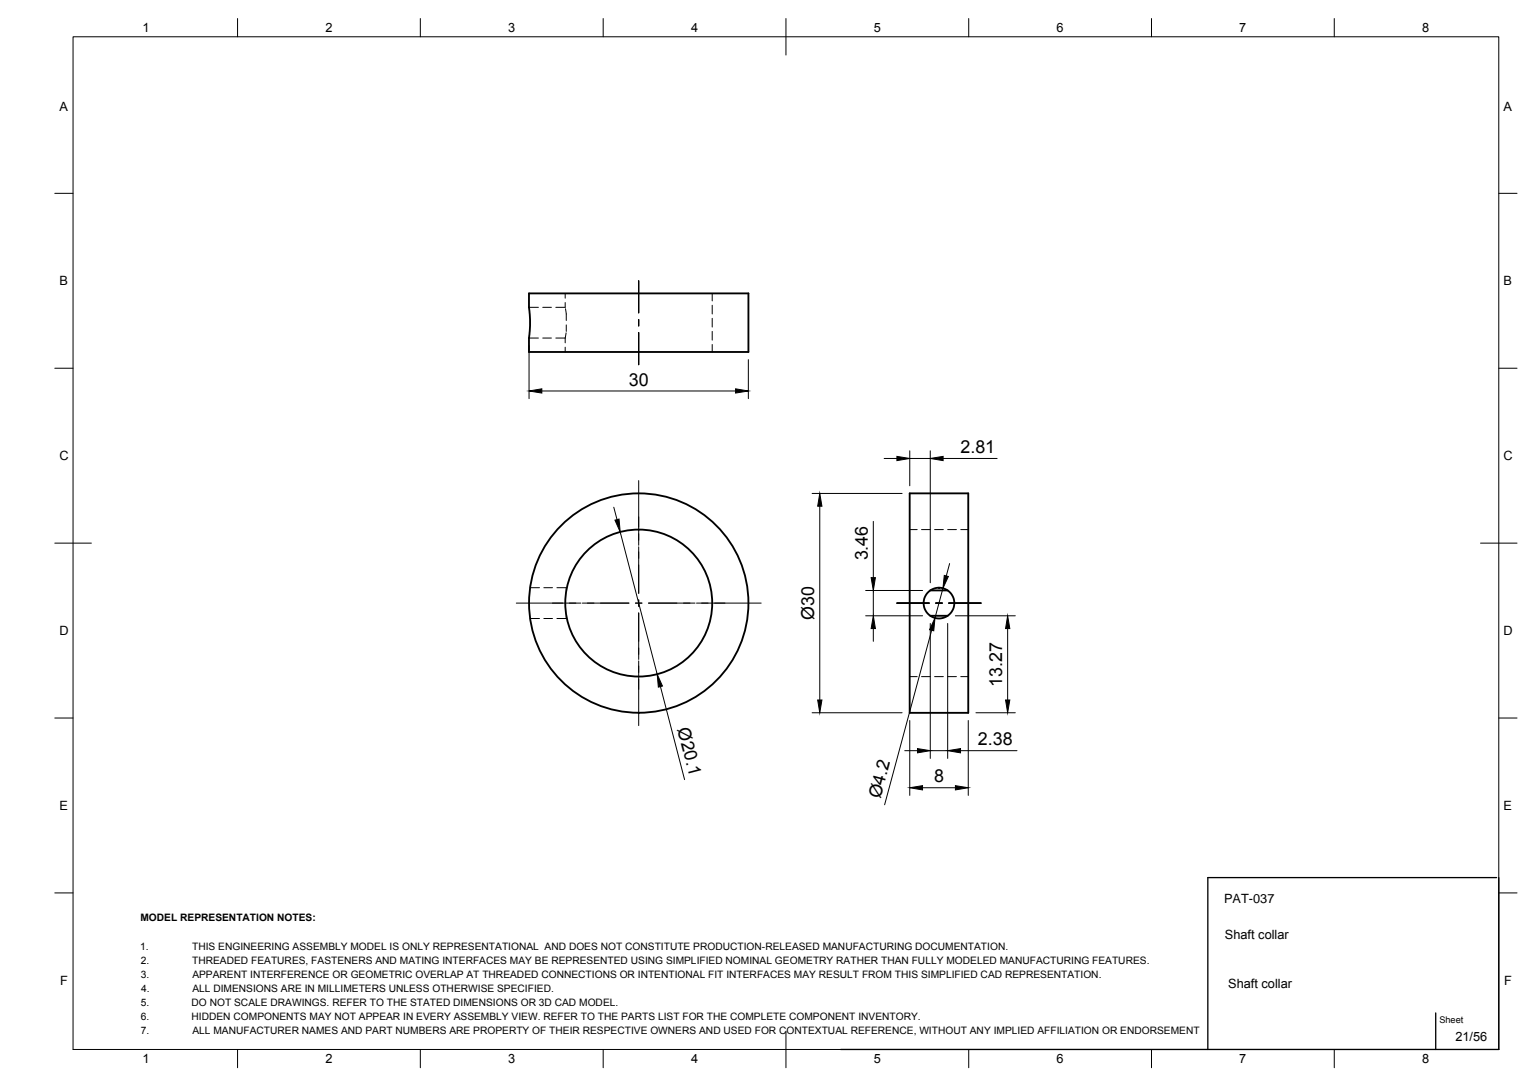
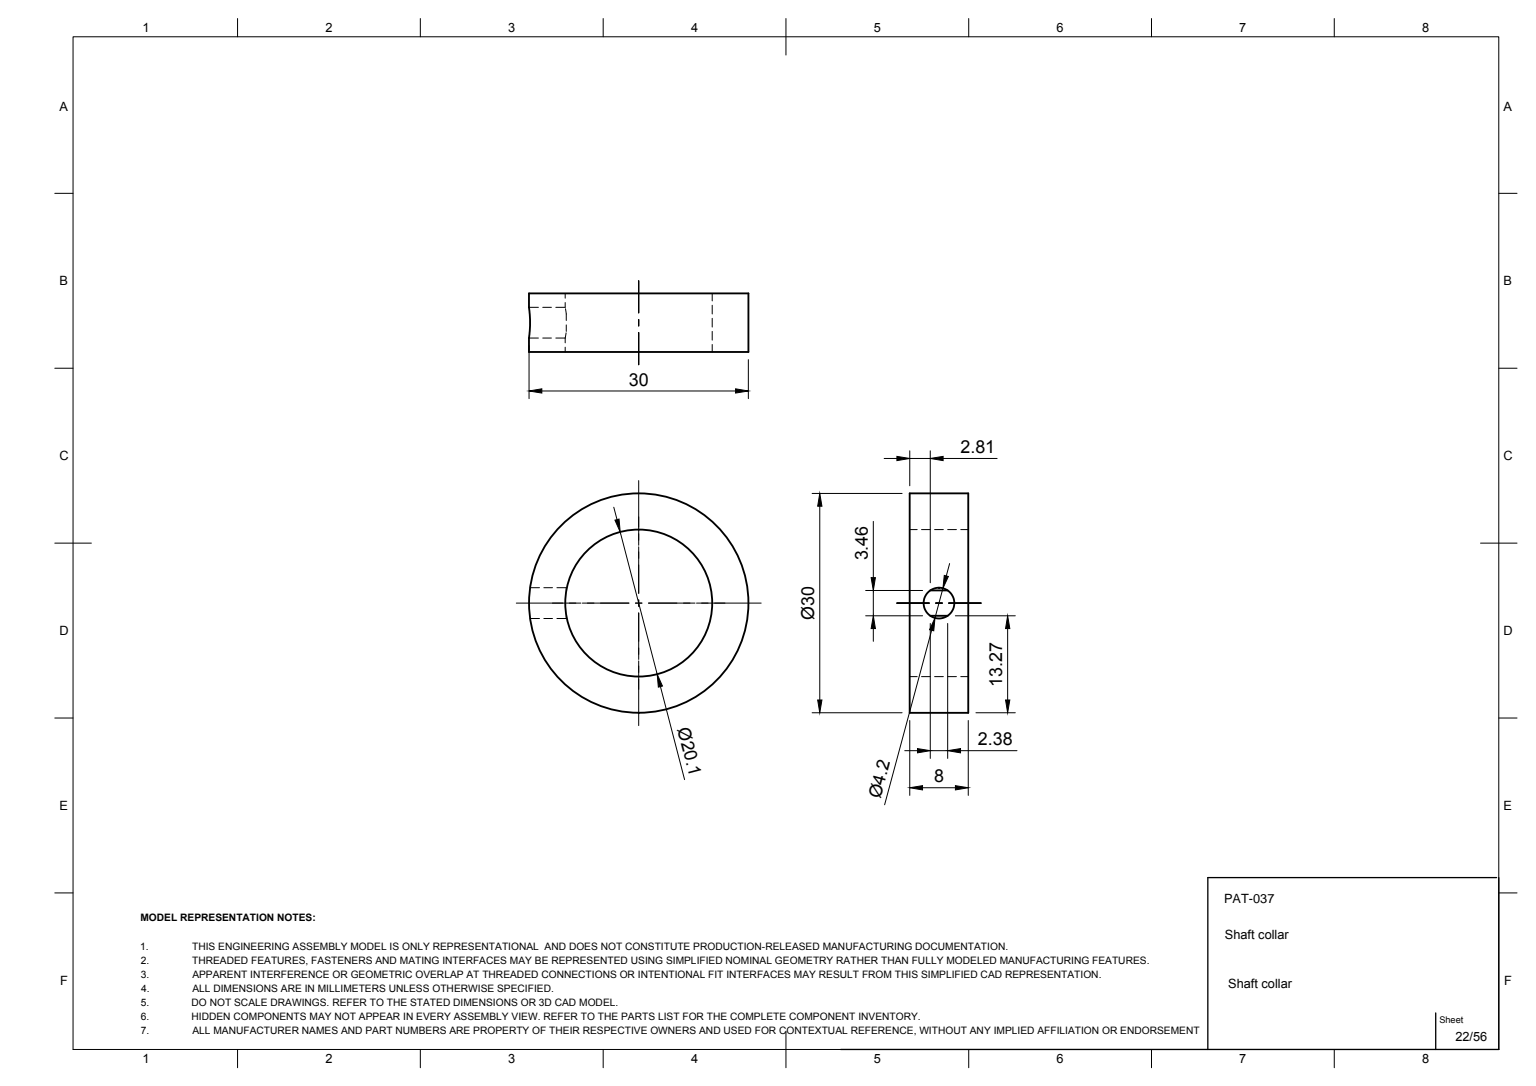
ISO-10303-21;
HEADER;
/* Generated by software containing ST-Developer
 * from STEP Tools, Inc. (www.steptools.com) 
 */

FILE_DESCRIPTION(
/* description */ ('Flywheel Crank-Slider'),
/* implementation_level */ '2;1');

FILE_NAME(
/* name */ 'Shaft collar.step',
/* time_stamp */ '2026-10-28T03:23:13-07:00',
/* author */ (''),
/* organization */ (''),
/* preprocessor_version */ 'ST-DEVELOPER v20.2',
/* originating_system */ 'Autodesk Translation Framework v15.17.0.0',
/* authorisation */ '');

FILE_SCHEMA (('AUTOMOTIVE_DESIGN { 1 0 10303 214 3 1 1 }'));
ENDSEC;

DATA;
#10=MECHANICAL_DESIGN_GEOMETRIC_PRESENTATION_REPRESENTATION('',(#691),#17322);
#481=B_SPLINE_CURVE_WITH_KNOTS('',3,(#15442,#15443,#15444,#15445,#15446,
#15447,#15448,#15449,#15450,#15451,#15452,#15453,#15454,#15455),
 .UNSPECIFIED.,.F.,.F.,(4,2,2,2,2,2,4),(0.756005737987026,0.793568827564645,
0.8729225200542,0.952276212543755,1.03162990503331,1.11098359752287,1.14854668710048),
 .UNSPECIFIED.);
#482=B_SPLINE_CURVE_WITH_KNOTS('',3,(#15461,#15462,#15463,#15464,#15465,
#15466,#15467,#15468,#15469,#15470,#15471,#15472,#15473,#15474,#15475,#15476,
#15477,#15478),.UNSPECIFIED.,.F.,.F.,(4,2,2,2,2,2,2,2,4),(0.,0.0792165807733624,
0.158433161546725,0.23764869707457,0.316864232602414,0.396079768130259,
0.475295303658103,0.554511884431466,0.633728465204828),.UNSPECIFIED.);
#483=B_SPLINE_CURVE_WITH_KNOTS('',3,(#15479,#15480,#15481,#15482,#15483,
#15484,#15485,#15486,#15487,#15488,#15489,#15490,#15491,#15492,#15493,#15494,
#15495,#15496),.UNSPECIFIED.,.F.,.F.,(4,2,2,2,2,2,2,2,4),(0.633728465204828,
0.712945045978191,0.792161626751553,0.871377162279398,0.950592697807242,
1.02980823333509,1.10902376886293,1.18824034963629,1.26745693040966),
 .UNSPECIFIED.);
#484=B_SPLINE_CURVE_WITH_KNOTS('',3,(#15499,#15500,#15501,#15502,#15503,
#15504,#15505,#15506,#15507,#15508,#15509,#15510,#15511,#15512),
 .UNSPECIFIED.,.F.,.F.,(4,2,2,2,2,2,4),(0.121154929624522,0.158718019202141,
0.238071711691697,0.317425404181252,0.396779096670807,0.476132789160362,
0.513695878737981),.UNSPECIFIED.);
#586=SHAPE_REPRESENTATION_RELATIONSHIP('SRR','None',#17584,#638);
#638=ADVANCED_BREP_SHAPE_REPRESENTATION('',(#748),#17288);
#691=STYLED_ITEM('',(#17931),#748);
#748=MANIFOLD_SOLID_BREP('Body1',#9073);
#908=FACE_BOUND('',#2264,.T.);
#909=FACE_BOUND('',#2266,.T.);
#910=FACE_BOUND('',#2268,.T.);
#911=FACE_BOUND('',#2270,.T.);
#1181=PLANE('',#10198);
#1182=PLANE('',#10203);
#1183=PLANE('',#10210);
#1184=PLANE('',#10211);
#1602=FACE_OUTER_BOUND('',#2260,.T.);
#1603=FACE_OUTER_BOUND('',#2261,.T.);
#1604=FACE_OUTER_BOUND('',#2262,.T.);
#1605=FACE_OUTER_BOUND('',#2263,.T.);
#1606=FACE_OUTER_BOUND('',#2265,.T.);
#1607=FACE_OUTER_BOUND('',#2267,.T.);
#1608=FACE_OUTER_BOUND('',#2269,.T.);
#2260=EDGE_LOOP('',(#7308,#7309));
#2261=EDGE_LOOP('',(#7310,#7311,#7312,#7313,#7314,#7315,#7316,#7317,#7318));
#2262=EDGE_LOOP('',(#7319,#7320,#7321));
#2263=EDGE_LOOP('',(#7322,#7323,#7324,#7325));
#2264=EDGE_LOOP('',(#7326,#7327,#7328,#7329));
#2265=EDGE_LOOP('',(#7330,#7331,#7332,#7333));
#2266=EDGE_LOOP('',(#7334,#7335));
#2267=EDGE_LOOP('',(#7336));
#2268=EDGE_LOOP('',(#7337));
#2269=EDGE_LOOP('',(#7338));
#2270=EDGE_LOOP('',(#7339));
#2983=LINE('',#15438,#3594);
#2984=LINE('',#15459,#3595);
#2985=LINE('',#15514,#3596);
#2986=LINE('',#15519,#3597);
#2987=LINE('',#15525,#3598);
#3594=VECTOR('',#12225,1.);
#3595=VECTOR('',#12232,0.21);
#3596=VECTOR('',#12237,1.);
#3597=VECTOR('',#12242,1.005);
#3598=VECTOR('',#12249,1.5);
#4040=CIRCLE('',#10199,0.21);
#4041=CIRCLE('',#10201,0.21);
#4042=CIRCLE('',#10202,0.21);
#4043=CIRCLE('',#10205,1.005);
#4044=CIRCLE('',#10206,1.005);
#4045=CIRCLE('',#10208,1.5);
#4046=CIRCLE('',#10209,1.5);
#4669=VERTEX_POINT('',#15436);
#4670=VERTEX_POINT('',#15437);
#4671=VERTEX_POINT('',#15441);
#4672=VERTEX_POINT('',#15456);
#4673=VERTEX_POINT('',#15458);
#4674=VERTEX_POINT('',#15460);
#4675=VERTEX_POINT('',#15497);
#4676=VERTEX_POINT('',#15516);
#4677=VERTEX_POINT('',#15518);
#4678=VERTEX_POINT('',#15522);
#4679=VERTEX_POINT('',#15524);
#5611=EDGE_CURVE('',#4669,#4670,#2983,.T.);
#5612=EDGE_CURVE('',#4669,#4670,#4040,.T.);
#5613=EDGE_CURVE('',#4671,#4669,#481,.T.);
#5614=EDGE_CURVE('',#4672,#4671,#4041,.T.);
#5615=EDGE_CURVE('',#4672,#4673,#2984,.T.);
#5616=EDGE_CURVE('',#4674,#4673,#482,.T.);
#5617=EDGE_CURVE('',#4673,#4674,#483,.T.);
#5618=EDGE_CURVE('',#4675,#4672,#4042,.T.);
#5619=EDGE_CURVE('',#4670,#4675,#484,.T.);
#5620=EDGE_CURVE('',#4675,#4671,#2985,.T.);
#5621=EDGE_CURVE('',#4676,#4676,#4043,.T.);
#5622=EDGE_CURVE('',#4676,#4677,#2986,.T.);
#5623=EDGE_CURVE('',#4677,#4677,#4044,.T.);
#5624=EDGE_CURVE('',#4678,#4678,#4045,.T.);
#5625=EDGE_CURVE('',#4678,#4679,#2987,.T.);
#5626=EDGE_CURVE('',#4679,#4679,#4046,.T.);
#7308=ORIENTED_EDGE('',*,*,#5611,.F.);
#7309=ORIENTED_EDGE('',*,*,#5612,.T.);
#7310=ORIENTED_EDGE('',*,*,#5613,.F.);
#7311=ORIENTED_EDGE('',*,*,#5614,.F.);
#7312=ORIENTED_EDGE('',*,*,#5615,.T.);
#7313=ORIENTED_EDGE('',*,*,#5616,.F.);
#7314=ORIENTED_EDGE('',*,*,#5617,.F.);
#7315=ORIENTED_EDGE('',*,*,#5615,.F.);
#7316=ORIENTED_EDGE('',*,*,#5618,.F.);
#7317=ORIENTED_EDGE('',*,*,#5619,.F.);
#7318=ORIENTED_EDGE('',*,*,#5612,.F.);
#7319=ORIENTED_EDGE('',*,*,#5620,.F.);
#7320=ORIENTED_EDGE('',*,*,#5618,.T.);
#7321=ORIENTED_EDGE('',*,*,#5614,.T.);
#7322=ORIENTED_EDGE('',*,*,#5621,.F.);
#7323=ORIENTED_EDGE('',*,*,#5622,.T.);
#7324=ORIENTED_EDGE('',*,*,#5623,.T.);
#7325=ORIENTED_EDGE('',*,*,#5622,.F.);
#7326=ORIENTED_EDGE('',*,*,#5619,.T.);
#7327=ORIENTED_EDGE('',*,*,#5620,.T.);
#7328=ORIENTED_EDGE('',*,*,#5613,.T.);
#7329=ORIENTED_EDGE('',*,*,#5611,.T.);
#7330=ORIENTED_EDGE('',*,*,#5624,.F.);
#7331=ORIENTED_EDGE('',*,*,#5625,.T.);
#7332=ORIENTED_EDGE('',*,*,#5626,.T.);
#7333=ORIENTED_EDGE('',*,*,#5625,.F.);
#7334=ORIENTED_EDGE('',*,*,#5616,.T.);
#7335=ORIENTED_EDGE('',*,*,#5617,.T.);
#7336=ORIENTED_EDGE('',*,*,#5624,.T.);
#7337=ORIENTED_EDGE('',*,*,#5621,.T.);
#7338=ORIENTED_EDGE('',*,*,#5626,.F.);
#7339=ORIENTED_EDGE('',*,*,#5623,.F.);
#8424=CYLINDRICAL_SURFACE('',#10200,0.21);
#8425=CYLINDRICAL_SURFACE('',#10204,1.005);
#8426=CYLINDRICAL_SURFACE('',#10207,1.5);
#8793=ADVANCED_FACE('',(#1602),#1181,.T.);
#8794=ADVANCED_FACE('',(#1603),#8424,.F.);
#8795=ADVANCED_FACE('',(#1604),#1182,.T.);
#8796=ADVANCED_FACE('',(#1605,#908),#8425,.F.);
#8797=ADVANCED_FACE('',(#1606,#909),#8426,.T.);
#8798=ADVANCED_FACE('',(#1607,#910),#1183,.T.);
#8799=ADVANCED_FACE('',(#1608,#911),#1184,.F.);
#9073=CLOSED_SHELL('',(#8793,#8794,#8795,#8796,#8797,#8798,#8799));
#10197=AXIS2_PLACEMENT_3D('',#15434,#12221,#12222);
#10198=AXIS2_PLACEMENT_3D('',#15435,#12223,#12224);
#10199=AXIS2_PLACEMENT_3D('',#15439,#12226,#12227);
#10200=AXIS2_PLACEMENT_3D('',#15440,#12228,#12229);
#10201=AXIS2_PLACEMENT_3D('',#15457,#12230,#12231);
#10202=AXIS2_PLACEMENT_3D('',#15498,#12233,#12234);
#10203=AXIS2_PLACEMENT_3D('',#15513,#12235,#12236);
#10204=AXIS2_PLACEMENT_3D('',#15515,#12238,#12239);
#10205=AXIS2_PLACEMENT_3D('',#15517,#12240,#12241);
#10206=AXIS2_PLACEMENT_3D('',#15520,#12243,#12244);
#10207=AXIS2_PLACEMENT_3D('',#15521,#12245,#12246);
#10208=AXIS2_PLACEMENT_3D('',#15523,#12247,#12248);
#10209=AXIS2_PLACEMENT_3D('',#15526,#12250,#12251);
#10210=AXIS2_PLACEMENT_3D('',#15527,#12252,#12253);
#10211=AXIS2_PLACEMENT_3D('',#15528,#12254,#12255);
#12221=DIRECTION('axis',(0.,0.,1.));
#12222=DIRECTION('refdir',(1.,0.,0.));
#12223=DIRECTION('center_axis',(0.,0.,1.));
#12224=DIRECTION('ref_axis',(1.,0.,0.));
#12225=DIRECTION('',(0.,1.,0.));
#12226=DIRECTION('center_axis',(0.,0.,1.));
#12227=DIRECTION('ref_axis',(1.,0.,0.));
#12228=DIRECTION('center_axis',(0.,0.,1.));
#12229=DIRECTION('ref_axis',(1.,0.,0.));
#12230=DIRECTION('center_axis',(0.,0.,1.));
#12231=DIRECTION('ref_axis',(1.,0.,0.));
#12232=DIRECTION('',(0.,0.,1.));
#12233=DIRECTION('center_axis',(0.,0.,1.));
#12234=DIRECTION('ref_axis',(1.,0.,0.));
#12235=DIRECTION('center_axis',(0.,0.,1.));
#12236=DIRECTION('ref_axis',(1.,0.,0.));
#12237=DIRECTION('',(0.,-1.,0.));
#12238=DIRECTION('center_axis',(0.,1.,0.));
#12239=DIRECTION('ref_axis',(1.,0.,0.));
#12240=DIRECTION('center_axis',(0.,-1.,0.));
#12241=DIRECTION('ref_axis',(1.,0.,0.));
#12242=DIRECTION('',(0.,-1.,0.));
#12243=DIRECTION('center_axis',(0.,-1.,0.));
#12244=DIRECTION('ref_axis',(1.,0.,0.));
#12245=DIRECTION('center_axis',(0.,1.,0.));
#12246=DIRECTION('ref_axis',(1.,0.,0.));
#12247=DIRECTION('center_axis',(0.,1.,0.));
#12248=DIRECTION('ref_axis',(1.,0.,0.));
#12249=DIRECTION('',(0.,-1.,0.));
#12250=DIRECTION('center_axis',(0.,1.,0.));
#12251=DIRECTION('ref_axis',(1.,0.,0.));
#12252=DIRECTION('center_axis',(0.,1.,0.));
#12253=DIRECTION('ref_axis',(1.,0.,0.));
#12254=DIRECTION('center_axis',(0.,1.,0.));
#12255=DIRECTION('ref_axis',(1.,0.,0.));
#15434=CARTESIAN_POINT('',(0.,0.,0.));
#15435=CARTESIAN_POINT('Origin',(0.,-17.05,10.99));
#15436=CARTESIAN_POINT('',(0.172988438920051,-17.1690588089979,10.99));
#15437=CARTESIAN_POINT('',(0.172988438920051,-16.9309411910021,10.99));
#15438=CARTESIAN_POINT('',(0.172988438920051,-17.45,10.99));
#15439=CARTESIAN_POINT('Origin',(0.,-17.05,10.99));
#15440=CARTESIAN_POINT('Origin',(0.,-17.05,10.99));
#15441=CARTESIAN_POINT('',(-0.172988438920051,-17.1690588089979,10.99));
#15442=CARTESIAN_POINT('Ctrl Pts',(-0.172988438920051,-17.1690588089979,
10.99));
#15443=CARTESIAN_POINT('Ctrl Pts',(-0.165594865311311,-17.1798014223953,
10.9912919219764));
#15444=CARTESIAN_POINT('Ctrl Pts',(-0.157297138725604,-17.1896877093727,
10.992653949439));
#15445=CARTESIAN_POINT('Ctrl Pts',(-0.129892073845076,-17.2170927742533,
10.9967480843909));
#15446=CARTESIAN_POINT('Ctrl Pts',(-0.106330167759284,-17.233242056333,
10.9996958932764));
#15447=CARTESIAN_POINT('Ctrl Pts',(-0.0546129046324093,-17.2546977939649,
11.0038502947236));
#15448=CARTESIAN_POINT('Ctrl Pts',(-0.0264512308298518,-17.26,11.005));
#15449=CARTESIAN_POINT('Ctrl Pts',(0.0264512308298517,-17.26,11.005));
#15450=CARTESIAN_POINT('Ctrl Pts',(0.0546129046324092,-17.2546977939649,
11.0038502947236));
#15451=CARTESIAN_POINT('Ctrl Pts',(0.106330167759284,-17.233242056333,10.9996958932764));
#15452=CARTESIAN_POINT('Ctrl Pts',(0.129892073845076,-17.2170927742533,
10.9967480843909));
#15453=CARTESIAN_POINT('Ctrl Pts',(0.157297138725603,-17.1896877093727,
10.992653949439));
#15454=CARTESIAN_POINT('Ctrl Pts',(0.16559486531131,-17.1798014223953,10.9912919219764));
#15455=CARTESIAN_POINT('Ctrl Pts',(0.17298843892005,-17.1690588089979,10.99));
#15456=CARTESIAN_POINT('',(-0.21,-17.05,10.99));
#15457=CARTESIAN_POINT('Origin',(0.,-17.05,10.99));
#15458=CARTESIAN_POINT('',(-0.21,-17.05,11.4852272553384));
#15459=CARTESIAN_POINT('',(-0.21,-17.05,10.99));
#15460=CARTESIAN_POINT('',(0.21,-17.05,11.4852272553384));
#15461=CARTESIAN_POINT('Ctrl Pts',(0.21,-17.05,11.4852272553384));
#15462=CARTESIAN_POINT('Ctrl Pts',(0.21,-17.0764055269245,11.4852272553384));
#15463=CARTESIAN_POINT('Ctrl Pts',(0.204715737269596,-17.1045470740907,
11.4860041595441));
#15464=CARTESIAN_POINT('Ctrl Pts',(0.183273763036332,-17.1562762689051,
11.4888007328232));
#15465=CARTESIAN_POINT('Ctrl Pts',(0.167117923970393,-17.179866924128,11.4907789715758));
#15466=CARTESIAN_POINT('Ctrl Pts',(0.129867169887369,-17.217117678211,11.4944848114133));
#15467=CARTESIAN_POINT('Ctrl Pts',(0.106276408305765,-17.2332737100014,
11.4964545565713));
#15468=CARTESIAN_POINT('Ctrl Pts',(0.0545468514058993,-17.2547158248262,
11.4992316551565));
#15469=CARTESIAN_POINT('Ctrl Pts',(0.0264051785092816,-17.26,11.5));
#15470=CARTESIAN_POINT('Ctrl Pts',(-0.0264051785092815,-17.26,11.5));
#15471=CARTESIAN_POINT('Ctrl Pts',(-0.054546851405899,-17.2547158248262,
11.4992316551565));
#15472=CARTESIAN_POINT('Ctrl Pts',(-0.106276408305765,-17.2332737100014,
11.4964545565713));
#15473=CARTESIAN_POINT('Ctrl Pts',(-0.129867169887368,-17.217117678211,
11.4944848114133));
#15474=CARTESIAN_POINT('Ctrl Pts',(-0.167117923970393,-17.179866924128,
11.4907789715758));
#15475=CARTESIAN_POINT('Ctrl Pts',(-0.183273763036332,-17.1562762689051,
11.4888007328232));
#15476=CARTESIAN_POINT('Ctrl Pts',(-0.204715737269596,-17.1045470740907,
11.4860041595441));
#15477=CARTESIAN_POINT('Ctrl Pts',(-0.21,-17.0764055269245,11.4852272553384));
#15478=CARTESIAN_POINT('Ctrl Pts',(-0.21,-17.05,11.4852272553384));
#15479=CARTESIAN_POINT('Ctrl Pts',(-0.21,-17.05,11.4852272553384));
#15480=CARTESIAN_POINT('Ctrl Pts',(-0.21,-17.0235944730756,11.4852272553384));
#15481=CARTESIAN_POINT('Ctrl Pts',(-0.204715737269596,-16.9954529259093,
11.4860041595441));
#15482=CARTESIAN_POINT('Ctrl Pts',(-0.183273763036332,-16.9437237310949,
11.4888007328232));
#15483=CARTESIAN_POINT('Ctrl Pts',(-0.167117923970393,-16.920133075872,
11.4907789715758));
#15484=CARTESIAN_POINT('Ctrl Pts',(-0.129867169887369,-16.882882321789,
11.4944848114133));
#15485=CARTESIAN_POINT('Ctrl Pts',(-0.106276408305765,-16.8667262899986,
11.4964545565713));
#15486=CARTESIAN_POINT('Ctrl Pts',(-0.0545468514058993,-16.8452841751738,
11.4992316551565));
#15487=CARTESIAN_POINT('Ctrl Pts',(-0.0264051785092816,-16.84,11.5));
#15488=CARTESIAN_POINT('Ctrl Pts',(0.0264051785092815,-16.84,11.5));
#15489=CARTESIAN_POINT('Ctrl Pts',(0.0545468514058992,-16.8452841751738,
11.4992316551565));
#15490=CARTESIAN_POINT('Ctrl Pts',(0.106276408305765,-16.8667262899986,
11.4964545565713));
#15491=CARTESIAN_POINT('Ctrl Pts',(0.129867169887368,-16.882882321789,11.4944848114133));
#15492=CARTESIAN_POINT('Ctrl Pts',(0.167117923970393,-16.920133075872,11.4907789715758));
#15493=CARTESIAN_POINT('Ctrl Pts',(0.183273763036332,-16.9437237310949,
11.4888007328232));
#15494=CARTESIAN_POINT('Ctrl Pts',(0.204715737269596,-16.9954529259093,
11.4860041595441));
#15495=CARTESIAN_POINT('Ctrl Pts',(0.21,-17.0235944730756,11.4852272553384));
#15496=CARTESIAN_POINT('Ctrl Pts',(0.21,-17.05,11.4852272553384));
#15497=CARTESIAN_POINT('',(-0.172988438920051,-16.9309411910021,10.99));
#15498=CARTESIAN_POINT('Origin',(0.,-17.05,10.99));
#15499=CARTESIAN_POINT('Ctrl Pts',(0.17298843892005,-16.9309411910021,10.99));
#15500=CARTESIAN_POINT('Ctrl Pts',(0.16559486531131,-16.9201985776047,10.9912919219764));
#15501=CARTESIAN_POINT('Ctrl Pts',(0.157297138725604,-16.9103122906273,
10.9926539494391));
#15502=CARTESIAN_POINT('Ctrl Pts',(0.129892073845076,-16.8829072257467,
10.9967480843909));
#15503=CARTESIAN_POINT('Ctrl Pts',(0.106330167759284,-16.8667579436671,
10.9996958932764));
#15504=CARTESIAN_POINT('Ctrl Pts',(0.0546129046324093,-16.8453022060351,
11.0038502947236));
#15505=CARTESIAN_POINT('Ctrl Pts',(0.0264512308298517,-16.84,11.005));
#15506=CARTESIAN_POINT('Ctrl Pts',(-0.0264512308298517,-16.84,11.005));
#15507=CARTESIAN_POINT('Ctrl Pts',(-0.054612904632409,-16.8453022060351,
11.0038502947236));
#15508=CARTESIAN_POINT('Ctrl Pts',(-0.106330167759284,-16.8667579436671,
10.9996958932764));
#15509=CARTESIAN_POINT('Ctrl Pts',(-0.129892073845076,-16.8829072257467,
10.9967480843909));
#15510=CARTESIAN_POINT('Ctrl Pts',(-0.157297138725604,-16.9103122906273,
10.992653949439));
#15511=CARTESIAN_POINT('Ctrl Pts',(-0.165594865311311,-16.9201985776047,
10.9912919219764));
#15512=CARTESIAN_POINT('Ctrl Pts',(-0.172988438920051,-16.9309411910021,
10.99));
#15513=CARTESIAN_POINT('Origin',(0.,-17.05,10.99));
#15514=CARTESIAN_POINT('',(-0.172988438920051,-17.45,10.99));
#15515=CARTESIAN_POINT('Origin',(0.,-17.45,10.));
#15516=CARTESIAN_POINT('',(-1.005,-16.65,10.));
#15517=CARTESIAN_POINT('Origin',(0.,-16.65,10.));
#15518=CARTESIAN_POINT('',(-1.005,-17.45,10.));
#15519=CARTESIAN_POINT('',(-1.005,-17.45,10.));
#15520=CARTESIAN_POINT('Origin',(0.,-17.45,10.));
#15521=CARTESIAN_POINT('Origin',(0.,-17.45,10.));
#15522=CARTESIAN_POINT('',(-1.5,-16.65,10.));
#15523=CARTESIAN_POINT('Origin',(0.,-16.65,10.));
#15524=CARTESIAN_POINT('',(-1.5,-17.45,10.));
#15525=CARTESIAN_POINT('',(-1.5,-17.45,10.));
#15526=CARTESIAN_POINT('Origin',(0.,-17.45,10.));
#15527=CARTESIAN_POINT('Origin',(0.,-16.65,10.));
#15528=CARTESIAN_POINT('Origin',(0.,-17.45,10.));
#17227=UNCERTAINTY_MEASURE_WITH_UNIT(LENGTH_MEASURE(0.001),#17323,
'DISTANCE_ACCURACY_VALUE',
'Maximum model space distance between geometric entities at asserted c
onnectivities');
#17261=UNCERTAINTY_MEASURE_WITH_UNIT(LENGTH_MEASURE(0.001),#17323,
'DISTANCE_ACCURACY_VALUE',
'Maximum model space distance between geometric entities at asserted c
onnectivities');
#17288=(
GEOMETRIC_REPRESENTATION_CONTEXT(3)
GLOBAL_UNCERTAINTY_ASSIGNED_CONTEXT((#17227))
GLOBAL_UNIT_ASSIGNED_CONTEXT((#17323,#17325,#17326))
REPRESENTATION_CONTEXT('','3D')
);
#17322=(
GEOMETRIC_REPRESENTATION_CONTEXT(3)
GLOBAL_UNCERTAINTY_ASSIGNED_CONTEXT((#17261))
GLOBAL_UNIT_ASSIGNED_CONTEXT((#17323,#17325,#17326))
REPRESENTATION_CONTEXT('','3D')
);
#17323=(
LENGTH_UNIT()
NAMED_UNIT(*)
SI_UNIT(.CENTI.,.METRE.)
);
#17325=(
NAMED_UNIT(*)
PLANE_ANGLE_UNIT()
SI_UNIT($,.RADIAN.)
);
#17326=(
NAMED_UNIT(*)
SI_UNIT($,.STERADIAN.)
SOLID_ANGLE_UNIT()
);
#17353=SHAPE_DEFINITION_REPRESENTATION(#17415,#17584);
#17415=PRODUCT_DEFINITION_SHAPE('',$,#17645);
#17584=SHAPE_REPRESENTATION('',(#10197),#17288);
#17618=PRODUCT_DEFINITION_CONTEXT('part definition',#17800,'design');
#17645=PRODUCT_DEFINITION('Shaft collar','Shaft collar',#17705,#17618);
#17705=PRODUCT_DEFINITION_FORMATION('',$,#17828);
#17800=APPLICATION_CONTEXT(
'Core Data for Automotive Mechanical Design Process');
#17801=PRODUCT_CONTEXT('part definition',#17800,'mechanical');
#17828=PRODUCT('Shaft collar','Shaft collar','Shaft collar',(#17801));
#17925=COLOUR_RGB('Grey',0.48,0.52,0.57);
#17926=FILL_AREA_STYLE_COLOUR('',#17925);
#17927=FILL_AREA_STYLE('',(#17926));
#17928=SURFACE_STYLE_FILL_AREA(#17927);
#17929=SURFACE_SIDE_STYLE('',(#17928));
#17930=SURFACE_STYLE_USAGE(.BOTH.,#17929);
#17931=PRESENTATION_STYLE_ASSIGNMENT((#17930));
ENDSEC;
END-ISO-10303-21;
